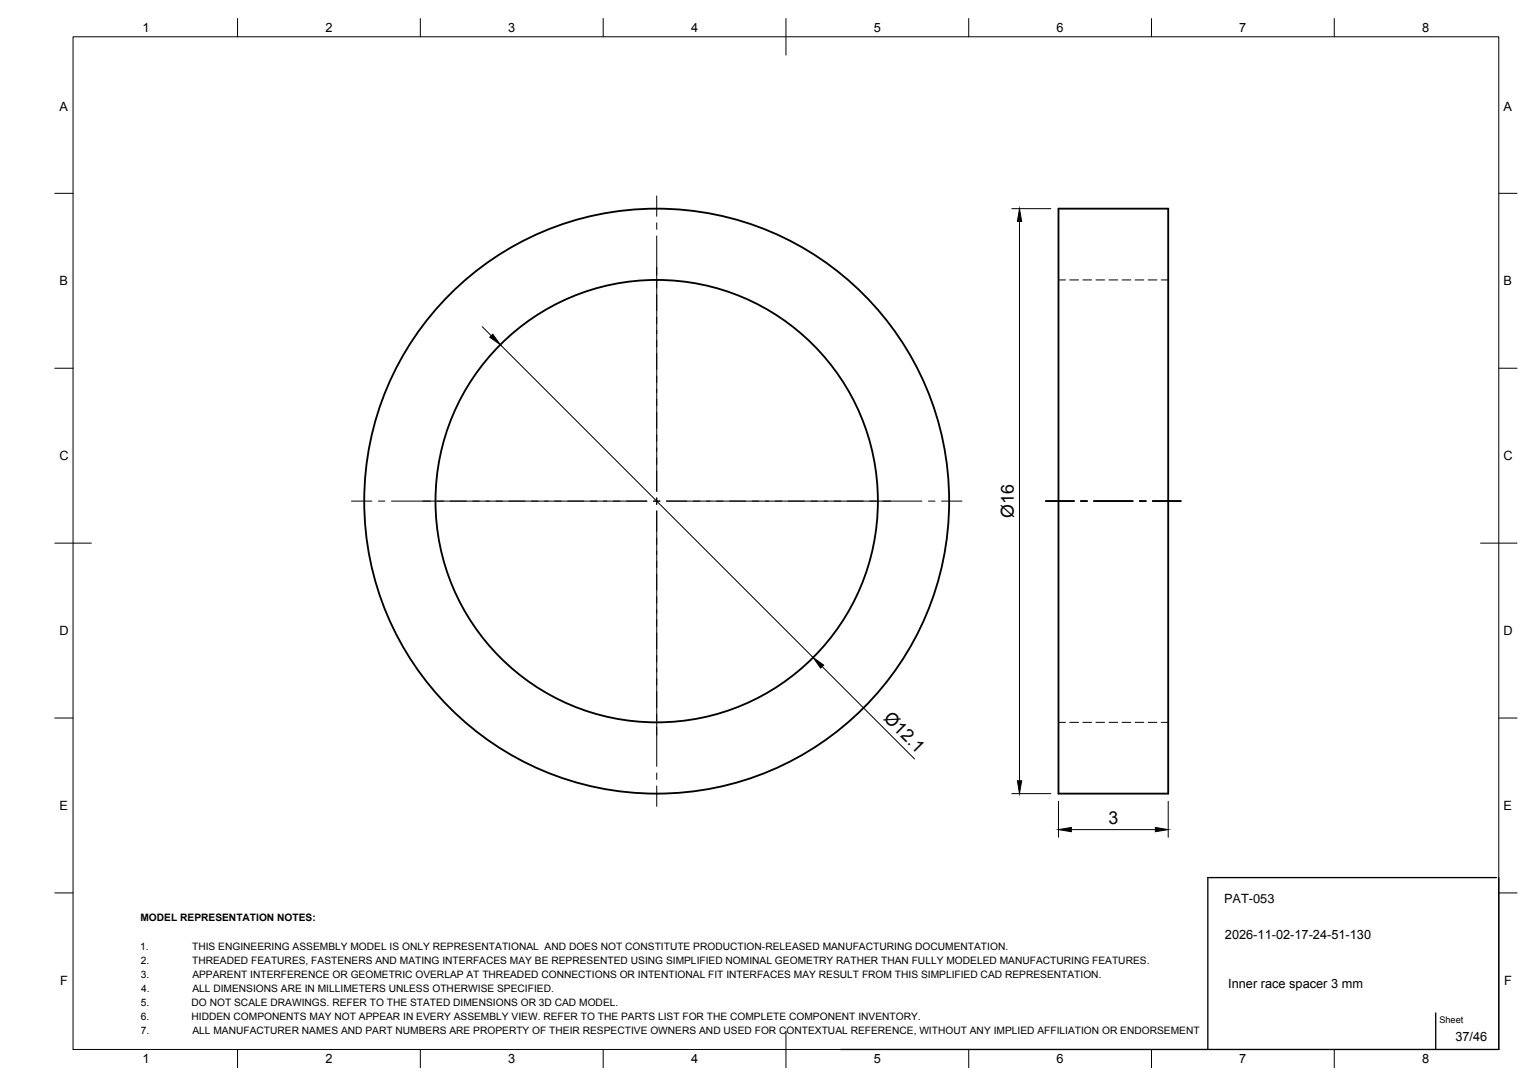
ISO-10303-21;
HEADER;
/* Generated by software containing ST-Developer
 * from STEP Tools, Inc. (www.steptools.com) 
 */

FILE_DESCRIPTION(
/* description */ ('Hand-operated arbor press'),
/* implementation_level */ '2;1');

FILE_NAME(
/* name */ 'Inner race spacer 3 mm.step',
/* time_stamp */ '2026-10-28T03:25:25-07:00',
/* author */ (''),
/* organization */ (''),
/* preprocessor_version */ 'ST-DEVELOPER v20.2',
/* originating_system */ 'Autodesk Translation Framework v15.17.0.0',
/* authorisation */ '');

FILE_SCHEMA (('AUTOMOTIVE_DESIGN { 1 0 10303 214 3 1 1 }'));
ENDSEC;

DATA;
#10=MECHANICAL_DESIGN_GEOMETRIC_PRESENTATION_REPRESENTATION('',(#622),#32751);
#531=SHAPE_REPRESENTATION_RELATIONSHIP('SRR','None',#32963,#573);
#573=ADVANCED_BREP_SHAPE_REPRESENTATION('',(#669),#32737);
#622=STYLED_ITEM('',(#33242),#669);
#669=MANIFOLD_SOLID_BREP('Body1',#12521);
#825=FACE_BOUND('',#2628,.T.);
#826=FACE_BOUND('',#2630,.T.);
#1210=PLANE('',#13847);
#1211=PLANE('',#13848);
#1799=FACE_OUTER_BOUND('',#2625,.T.);
#1800=FACE_OUTER_BOUND('',#2626,.T.);
#1801=FACE_OUTER_BOUND('',#2627,.T.);
#1802=FACE_OUTER_BOUND('',#2629,.T.);
#2625=EDGE_LOOP('',(#10812,#10813,#10814,#10815));
#2626=EDGE_LOOP('',(#10816,#10817,#10818,#10819));
#2627=EDGE_LOOP('',(#10820));
#2628=EDGE_LOOP('',(#10821));
#2629=EDGE_LOOP('',(#10822));
#2630=EDGE_LOOP('',(#10823));
#3758=LINE('',#20633,#4929);
#3759=LINE('',#20639,#4930);
#4929=VECTOR('',#16777,0.605);
#4930=VECTOR('',#16784,0.8);
#5458=CIRCLE('',#13842,0.605);
#5459=CIRCLE('',#13843,0.605);
#5460=CIRCLE('',#13845,0.8);
#5461=CIRCLE('',#13846,0.8);
#6391=VERTEX_POINT('',#20630);
#6392=VERTEX_POINT('',#20632);
#6393=VERTEX_POINT('',#20636);
#6394=VERTEX_POINT('',#20638);
#7909=EDGE_CURVE('',#6391,#6391,#5458,.T.);
#7910=EDGE_CURVE('',#6391,#6392,#3758,.T.);
#7911=EDGE_CURVE('',#6392,#6392,#5459,.T.);
#7912=EDGE_CURVE('',#6393,#6393,#5460,.T.);
#7913=EDGE_CURVE('',#6393,#6394,#3759,.T.);
#7914=EDGE_CURVE('',#6394,#6394,#5461,.T.);
#10812=ORIENTED_EDGE('',*,*,#7909,.F.);
#10813=ORIENTED_EDGE('',*,*,#7910,.T.);
#10814=ORIENTED_EDGE('',*,*,#7911,.T.);
#10815=ORIENTED_EDGE('',*,*,#7910,.F.);
#10816=ORIENTED_EDGE('',*,*,#7912,.F.);
#10817=ORIENTED_EDGE('',*,*,#7913,.T.);
#10818=ORIENTED_EDGE('',*,*,#7914,.T.);
#10819=ORIENTED_EDGE('',*,*,#7913,.F.);
#10820=ORIENTED_EDGE('',*,*,#7912,.T.);
#10821=ORIENTED_EDGE('',*,*,#7909,.T.);
#10822=ORIENTED_EDGE('',*,*,#7914,.F.);
#10823=ORIENTED_EDGE('',*,*,#7911,.F.);
#11758=CYLINDRICAL_SURFACE('',#13841,0.605);
#11759=CYLINDRICAL_SURFACE('',#13844,0.8);
#12308=ADVANCED_FACE('',(#1799),#11758,.F.);
#12309=ADVANCED_FACE('',(#1800),#11759,.T.);
#12310=ADVANCED_FACE('',(#1801,#825),#1210,.T.);
#12311=ADVANCED_FACE('',(#1802,#826),#1211,.F.);
#12521=CLOSED_SHELL('',(#12308,#12309,#12310,#12311));
#13840=AXIS2_PLACEMENT_3D('',#20628,#16771,#16772);
#13841=AXIS2_PLACEMENT_3D('',#20629,#16773,#16774);
#13842=AXIS2_PLACEMENT_3D('',#20631,#16775,#16776);
#13843=AXIS2_PLACEMENT_3D('',#20634,#16778,#16779);
#13844=AXIS2_PLACEMENT_3D('',#20635,#16780,#16781);
#13845=AXIS2_PLACEMENT_3D('',#20637,#16782,#16783);
#13846=AXIS2_PLACEMENT_3D('',#20640,#16785,#16786);
#13847=AXIS2_PLACEMENT_3D('',#20641,#16787,#16788);
#13848=AXIS2_PLACEMENT_3D('',#20642,#16789,#16790);
#16771=DIRECTION('axis',(0.,0.,1.));
#16772=DIRECTION('refdir',(1.,0.,0.));
#16773=DIRECTION('center_axis',(0.,1.,0.));
#16774=DIRECTION('ref_axis',(1.,0.,0.));
#16775=DIRECTION('center_axis',(0.,-1.,0.));
#16776=DIRECTION('ref_axis',(1.,0.,0.));
#16777=DIRECTION('',(0.,-1.,0.));
#16778=DIRECTION('center_axis',(0.,-1.,0.));
#16779=DIRECTION('ref_axis',(1.,0.,0.));
#16780=DIRECTION('center_axis',(0.,1.,0.));
#16781=DIRECTION('ref_axis',(1.,0.,0.));
#16782=DIRECTION('center_axis',(0.,1.,0.));
#16783=DIRECTION('ref_axis',(1.,0.,0.));
#16784=DIRECTION('',(0.,-1.,0.));
#16785=DIRECTION('center_axis',(0.,1.,0.));
#16786=DIRECTION('ref_axis',(1.,0.,0.));
#16787=DIRECTION('center_axis',(0.,1.,0.));
#16788=DIRECTION('ref_axis',(1.,0.,0.));
#16789=DIRECTION('center_axis',(0.,1.,0.));
#16790=DIRECTION('ref_axis',(1.,0.,0.));
#20628=CARTESIAN_POINT('',(0.,0.,0.));
#20629=CARTESIAN_POINT('Origin',(-3.25,2.2,20.));
#20630=CARTESIAN_POINT('',(-3.855,2.5,20.));
#20631=CARTESIAN_POINT('Origin',(-3.25,2.5,20.));
#20632=CARTESIAN_POINT('',(-3.855,2.2,20.));
#20633=CARTESIAN_POINT('',(-3.855,2.2,20.));
#20634=CARTESIAN_POINT('Origin',(-3.25,2.2,20.));
#20635=CARTESIAN_POINT('Origin',(-3.25,2.2,20.));
#20636=CARTESIAN_POINT('',(-4.05,2.5,20.));
#20637=CARTESIAN_POINT('Origin',(-3.25,2.5,20.));
#20638=CARTESIAN_POINT('',(-4.05,2.2,20.));
#20639=CARTESIAN_POINT('',(-4.05,2.2,20.));
#20640=CARTESIAN_POINT('Origin',(-3.25,2.2,20.));
#20641=CARTESIAN_POINT('Origin',(-3.25,2.5,20.));
#20642=CARTESIAN_POINT('Origin',(-3.25,2.2,20.));
#32688=UNCERTAINTY_MEASURE_WITH_UNIT(LENGTH_MEASURE(0.001),#32752,
'DISTANCE_ACCURACY_VALUE',
'Maximum model space distance between geometric entities at asserted c
onnectivities');
#32702=UNCERTAINTY_MEASURE_WITH_UNIT(LENGTH_MEASURE(0.001),#32752,
'DISTANCE_ACCURACY_VALUE',
'Maximum model space distance between geometric entities at asserted c
onnectivities');
#32737=(
GEOMETRIC_REPRESENTATION_CONTEXT(3)
GLOBAL_UNCERTAINTY_ASSIGNED_CONTEXT((#32688))
GLOBAL_UNIT_ASSIGNED_CONTEXT((#32752,#32754,#32755))
REPRESENTATION_CONTEXT('','3D')
);
#32751=(
GEOMETRIC_REPRESENTATION_CONTEXT(3)
GLOBAL_UNCERTAINTY_ASSIGNED_CONTEXT((#32702))
GLOBAL_UNIT_ASSIGNED_CONTEXT((#32752,#32754,#32755))
REPRESENTATION_CONTEXT('','3D')
);
#32752=(
LENGTH_UNIT()
NAMED_UNIT(*)
SI_UNIT(.CENTI.,.METRE.)
);
#32754=(
NAMED_UNIT(*)
PLANE_ANGLE_UNIT()
SI_UNIT($,.RADIAN.)
);
#32755=(
NAMED_UNIT(*)
SI_UNIT($,.STERADIAN.)
SOLID_ANGLE_UNIT()
);
#32790=SHAPE_DEFINITION_REPRESENTATION(#32847,#32963);
#32847=PRODUCT_DEFINITION_SHAPE('',$,#33012);
#32963=SHAPE_REPRESENTATION('',(#13840),#32737);
#32977=PRODUCT_DEFINITION_CONTEXT('part definition',#33123,'design');
#33012=PRODUCT_DEFINITION('Inner race spacer 3 mm',
'Inner race spacer 3 mm',#33060,#32977);
#33060=PRODUCT_DEFINITION_FORMATION('',$,#33159);
#33123=APPLICATION_CONTEXT(
'Core Data for Automotive Mechanical Design Process');
#33124=PRODUCT_CONTEXT('part definition',#33123,'mechanical');
#33159=PRODUCT('Inner race spacer 3 mm','Inner race spacer 3 mm',
'Inner race spacer 3 mm',(#33124));
#33236=COLOUR_RGB('Grey',0.48,0.52,0.57);
#33237=FILL_AREA_STYLE_COLOUR('',#33236);
#33238=FILL_AREA_STYLE('',(#33237));
#33239=SURFACE_STYLE_FILL_AREA(#33238);
#33240=SURFACE_SIDE_STYLE('',(#33239));
#33241=SURFACE_STYLE_USAGE(.BOTH.,#33240);
#33242=PRESENTATION_STYLE_ASSIGNMENT((#33241));
ENDSEC;
END-ISO-10303-21;
